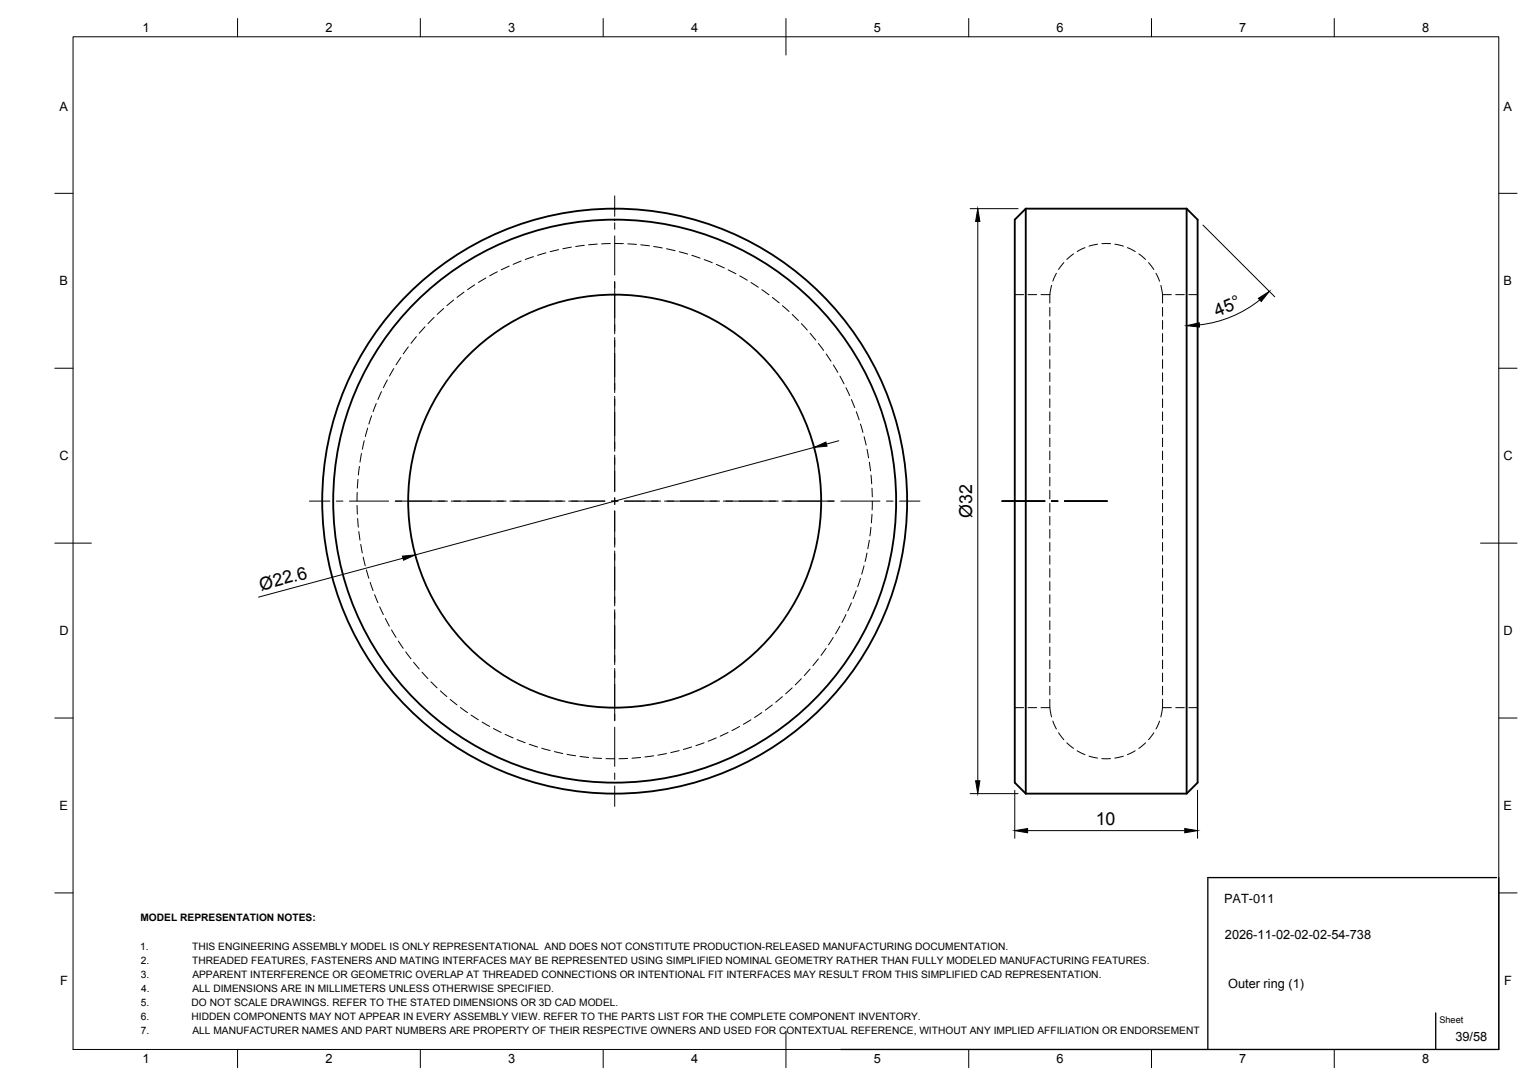
ISO-10303-21;
HEADER;
/* Generated by software containing ST-Developer
 * from STEP Tools, Inc. (www.steptools.com) 
 */

FILE_DESCRIPTION(
/* description */ ('Belt tension measurement rig'),
/* implementation_level */ '2;1');

FILE_NAME(
/* name */ 'Outer ring (1).step',
/* time_stamp */ '2026-10-28T03:24:44-07:00',
/* author */ (''),
/* organization */ (''),
/* preprocessor_version */ 'ST-DEVELOPER v20.2',
/* originating_system */ 'Autodesk Translation Framework v15.17.0.0',
/* authorisation */ '');

FILE_SCHEMA (('AUTOMOTIVE_DESIGN { 1 0 10303 214 3 1 1 }'));
ENDSEC;

DATA;
#10=MECHANICAL_DESIGN_GEOMETRIC_PRESENTATION_REPRESENTATION('',(#732),#23587);
#476=CONICAL_SURFACE('',#13686,1.57,0.785398163397449);
#477=CONICAL_SURFACE('',#13690,1.57,0.785398163397449);
#490=TOROIDAL_SURFACE('',#13675,1.1,0.309556);
#614=SHAPE_REPRESENTATION_RELATIONSHIP('SRR','None',#23863,#669);
#669=ADVANCED_BREP_SHAPE_REPRESENTATION('',(#801),#23561);
#732=STYLED_ITEM('',(#24211),#801);
#801=MANIFOLD_SOLID_BREP('Body1',#12238);
#976=FACE_BOUND('',#2597,.T.);
#977=FACE_BOUND('',#2602,.T.);
#1252=PLANE('',#13683);
#1253=PLANE('',#13692);
#1743=FACE_OUTER_BOUND('',#2594,.T.);
#1744=FACE_OUTER_BOUND('',#2595,.T.);
#1745=FACE_OUTER_BOUND('',#2596,.T.);
#1746=FACE_OUTER_BOUND('',#2598,.T.);
#1747=FACE_OUTER_BOUND('',#2599,.T.);
#1748=FACE_OUTER_BOUND('',#2600,.T.);
#1749=FACE_OUTER_BOUND('',#2601,.T.);
#1750=FACE_OUTER_BOUND('',#2603,.T.);
#2594=EDGE_LOOP('',(#9694,#9695,#9696,#9697,#9698,#9699));
#2595=EDGE_LOOP('',(#9700,#9701,#9702,#9703,#9704));
#2596=EDGE_LOOP('',(#9705));
#2597=EDGE_LOOP('',(#9706));
#2598=EDGE_LOOP('',(#9707,#9708,#9709,#9710));
#2599=EDGE_LOOP('',(#9711,#9712,#9713,#9714));
#2600=EDGE_LOOP('',(#9715,#9716,#9717,#9718));
#2601=EDGE_LOOP('',(#9719));
#2602=EDGE_LOOP('',(#9720));
#2603=EDGE_LOOP('',(#9721,#9722,#9723,#9724,#9725));
#3459=LINE('',#20899,#4210);
#3460=LINE('',#20908,#4211);
#3461=LINE('',#20912,#4212);
#3462=LINE('',#20916,#4213);
#3463=LINE('',#20919,#4214);
#4210=VECTOR('',#16622,1.129765);
#4211=VECTOR('',#16633,1.57);
#4212=VECTOR('',#16638,1.6);
#4213=VECTOR('',#16643,1.57);
#4214=VECTOR('',#16648,1.129765);
#4831=CIRCLE('',#13676,1.129765);
#4832=CIRCLE('',#13677,1.129765);
#4833=CIRCLE('',#13678,0.309556);
#4834=CIRCLE('',#13679,1.129765);
#4835=CIRCLE('',#13680,1.129765);
#4836=CIRCLE('',#13682,1.129765);
#4837=CIRCLE('',#13684,1.54);
#4838=CIRCLE('',#13685,1.129765);
#4839=CIRCLE('',#13687,1.6);
#4840=CIRCLE('',#13689,1.6);
#4841=CIRCLE('',#13691,1.54);
#5828=VERTEX_POINT('',#20887);
#5829=VERTEX_POINT('',#20888);
#5830=VERTEX_POINT('',#20891);
#5831=VERTEX_POINT('',#20893);
#5832=VERTEX_POINT('',#20897);
#5833=VERTEX_POINT('',#20901);
#5834=VERTEX_POINT('',#20903);
#5835=VERTEX_POINT('',#20906);
#5836=VERTEX_POINT('',#20910);
#5837=VERTEX_POINT('',#20914);
#7206=EDGE_CURVE('',#5828,#5829,#4831,.T.);
#7207=EDGE_CURVE('',#5829,#5828,#4832,.T.);
#7208=EDGE_CURVE('',#5829,#5830,#4833,.T.);
#7209=EDGE_CURVE('',#5831,#5830,#4834,.T.);
#7210=EDGE_CURVE('',#5830,#5831,#4835,.T.);
#7211=EDGE_CURVE('',#5832,#5832,#4836,.T.);
#7212=EDGE_CURVE('',#5832,#5831,#3459,.T.);
#7213=EDGE_CURVE('',#5833,#5833,#4837,.T.);
#7214=EDGE_CURVE('',#5834,#5834,#4838,.T.);
#7215=EDGE_CURVE('',#5835,#5835,#4839,.T.);
#7216=EDGE_CURVE('',#5835,#5833,#3460,.T.);
#7217=EDGE_CURVE('',#5836,#5836,#4840,.T.);
#7218=EDGE_CURVE('',#5836,#5835,#3461,.T.);
#7219=EDGE_CURVE('',#5837,#5837,#4841,.T.);
#7220=EDGE_CURVE('',#5837,#5836,#3462,.T.);
#7221=EDGE_CURVE('',#5828,#5834,#3463,.T.);
#9694=ORIENTED_EDGE('',*,*,#7206,.F.);
#9695=ORIENTED_EDGE('',*,*,#7207,.F.);
#9696=ORIENTED_EDGE('',*,*,#7208,.T.);
#9697=ORIENTED_EDGE('',*,*,#7209,.F.);
#9698=ORIENTED_EDGE('',*,*,#7210,.F.);
#9699=ORIENTED_EDGE('',*,*,#7208,.F.);
#9700=ORIENTED_EDGE('',*,*,#7211,.T.);
#9701=ORIENTED_EDGE('',*,*,#7212,.T.);
#9702=ORIENTED_EDGE('',*,*,#7209,.T.);
#9703=ORIENTED_EDGE('',*,*,#7210,.T.);
#9704=ORIENTED_EDGE('',*,*,#7212,.F.);
#9705=ORIENTED_EDGE('',*,*,#7213,.F.);
#9706=ORIENTED_EDGE('',*,*,#7214,.T.);
#9707=ORIENTED_EDGE('',*,*,#7215,.F.);
#9708=ORIENTED_EDGE('',*,*,#7216,.T.);
#9709=ORIENTED_EDGE('',*,*,#7213,.T.);
#9710=ORIENTED_EDGE('',*,*,#7216,.F.);
#9711=ORIENTED_EDGE('',*,*,#7217,.F.);
#9712=ORIENTED_EDGE('',*,*,#7218,.T.);
#9713=ORIENTED_EDGE('',*,*,#7215,.T.);
#9714=ORIENTED_EDGE('',*,*,#7218,.F.);
#9715=ORIENTED_EDGE('',*,*,#7219,.F.);
#9716=ORIENTED_EDGE('',*,*,#7220,.T.);
#9717=ORIENTED_EDGE('',*,*,#7217,.T.);
#9718=ORIENTED_EDGE('',*,*,#7220,.F.);
#9719=ORIENTED_EDGE('',*,*,#7219,.T.);
#9720=ORIENTED_EDGE('',*,*,#7211,.F.);
#9721=ORIENTED_EDGE('',*,*,#7206,.T.);
#9722=ORIENTED_EDGE('',*,*,#7207,.T.);
#9723=ORIENTED_EDGE('',*,*,#7221,.T.);
#9724=ORIENTED_EDGE('',*,*,#7214,.F.);
#9725=ORIENTED_EDGE('',*,*,#7221,.F.);
#11306=CYLINDRICAL_SURFACE('',#13681,1.129765);
#11307=CYLINDRICAL_SURFACE('',#13688,1.6);
#11308=CYLINDRICAL_SURFACE('',#13693,1.129765);
#11884=ADVANCED_FACE('',(#1743),#490,.F.);
#11885=ADVANCED_FACE('',(#1744),#11306,.F.);
#11886=ADVANCED_FACE('',(#1745,#976),#1252,.T.);
#11887=ADVANCED_FACE('',(#1746),#476,.T.);
#11888=ADVANCED_FACE('',(#1747),#11307,.T.);
#11889=ADVANCED_FACE('',(#1748),#477,.T.);
#11890=ADVANCED_FACE('',(#1749,#977),#1253,.T.);
#11891=ADVANCED_FACE('',(#1750),#11308,.F.);
#12238=CLOSED_SHELL('',(#11884,#11885,#11886,#11887,#11888,#11889,#11890,
#11891));
#13674=AXIS2_PLACEMENT_3D('',#20885,#16604,#16605);
#13675=AXIS2_PLACEMENT_3D('',#20886,#16606,#16607);
#13676=AXIS2_PLACEMENT_3D('',#20889,#16608,#16609);
#13677=AXIS2_PLACEMENT_3D('',#20890,#16610,#16611);
#13678=AXIS2_PLACEMENT_3D('',#20892,#16612,#16613);
#13679=AXIS2_PLACEMENT_3D('',#20894,#16614,#16615);
#13680=AXIS2_PLACEMENT_3D('',#20895,#16616,#16617);
#13681=AXIS2_PLACEMENT_3D('',#20896,#16618,#16619);
#13682=AXIS2_PLACEMENT_3D('',#20898,#16620,#16621);
#13683=AXIS2_PLACEMENT_3D('',#20900,#16623,#16624);
#13684=AXIS2_PLACEMENT_3D('',#20902,#16625,#16626);
#13685=AXIS2_PLACEMENT_3D('',#20904,#16627,#16628);
#13686=AXIS2_PLACEMENT_3D('',#20905,#16629,#16630);
#13687=AXIS2_PLACEMENT_3D('',#20907,#16631,#16632);
#13688=AXIS2_PLACEMENT_3D('',#20909,#16634,#16635);
#13689=AXIS2_PLACEMENT_3D('',#20911,#16636,#16637);
#13690=AXIS2_PLACEMENT_3D('',#20913,#16639,#16640);
#13691=AXIS2_PLACEMENT_3D('',#20915,#16641,#16642);
#13692=AXIS2_PLACEMENT_3D('',#20917,#16644,#16645);
#13693=AXIS2_PLACEMENT_3D('',#20918,#16646,#16647);
#16604=DIRECTION('axis',(0.,0.,1.));
#16605=DIRECTION('refdir',(1.,0.,0.));
#16606=DIRECTION('center_axis',(0.,-1.,0.));
#16607=DIRECTION('ref_axis',(0.,0.,-1.));
#16608=DIRECTION('center_axis',(0.,-1.,0.));
#16609=DIRECTION('ref_axis',(1.,0.,0.));
#16610=DIRECTION('center_axis',(0.,-1.,0.));
#16611=DIRECTION('ref_axis',(1.,0.,0.));
#16612=DIRECTION('center_axis',(1.,0.,1.22464679914735E-16));
#16613=DIRECTION('ref_axis',(-1.22464679914735E-16,0.,1.));
#16614=DIRECTION('center_axis',(0.,1.,0.));
#16615=DIRECTION('ref_axis',(1.,0.,0.));
#16616=DIRECTION('center_axis',(0.,1.,0.));
#16617=DIRECTION('ref_axis',(1.,0.,0.));
#16618=DIRECTION('center_axis',(0.,-1.,0.));
#16619=DIRECTION('ref_axis',(1.,0.,0.));
#16620=DIRECTION('center_axis',(0.,-1.,0.));
#16621=DIRECTION('ref_axis',(1.,0.,0.));
#16622=DIRECTION('',(0.,1.,0.));
#16623=DIRECTION('center_axis',(0.,1.,0.));
#16624=DIRECTION('ref_axis',(0.,0.,1.));
#16625=DIRECTION('center_axis',(0.,-1.,0.));
#16626=DIRECTION('ref_axis',(1.,0.,0.));
#16627=DIRECTION('center_axis',(0.,-1.,0.));
#16628=DIRECTION('ref_axis',(1.,0.,0.));
#16629=DIRECTION('center_axis',(0.,-1.,0.));
#16630=DIRECTION('ref_axis',(1.,0.,0.));
#16631=DIRECTION('center_axis',(0.,-1.,0.));
#16632=DIRECTION('ref_axis',(1.,0.,0.));
#16633=DIRECTION('',(0.707106781186548,0.707106781186547,8.65956056235494E-17));
#16634=DIRECTION('center_axis',(0.,-1.,0.));
#16635=DIRECTION('ref_axis',(1.,0.,0.));
#16636=DIRECTION('center_axis',(0.,-1.,0.));
#16637=DIRECTION('ref_axis',(1.,0.,0.));
#16638=DIRECTION('',(0.,1.,0.));
#16639=DIRECTION('center_axis',(0.,1.,0.));
#16640=DIRECTION('ref_axis',(1.,0.,0.));
#16641=DIRECTION('center_axis',(0.,-1.,0.));
#16642=DIRECTION('ref_axis',(1.,0.,0.));
#16643=DIRECTION('',(-0.707106781186548,0.707106781186547,-8.65956056235494E-17));
#16644=DIRECTION('center_axis',(0.,-1.,0.));
#16645=DIRECTION('ref_axis',(0.,0.,-1.));
#16646=DIRECTION('center_axis',(0.,-1.,0.));
#16647=DIRECTION('ref_axis',(1.,0.,0.));
#16648=DIRECTION('',(0.,1.,0.));
#20885=CARTESIAN_POINT('',(0.,0.,0.));
#20886=CARTESIAN_POINT('Origin',(0.,0.,0.));
#20887=CARTESIAN_POINT('',(-1.129765,0.308121667383195,-1.38356309103871E-16));
#20888=CARTESIAN_POINT('',(-1.38356309103871E-16,0.308121667383195,1.129765));
#20889=CARTESIAN_POINT('Origin',(0.,0.308121667383195,0.));
#20890=CARTESIAN_POINT('Origin',(0.,0.308121667383195,0.));
#20891=CARTESIAN_POINT('',(-1.38356309103871E-16,-0.308121667383195,1.129765));
#20892=CARTESIAN_POINT('Origin',(-1.34711147906209E-16,0.,1.1));
#20893=CARTESIAN_POINT('',(-1.129765,-0.308121667383195,1.38356309103871E-16));
#20894=CARTESIAN_POINT('Origin',(0.,-0.308121667383195,0.));
#20895=CARTESIAN_POINT('Origin',(0.,-0.308121667383195,0.));
#20896=CARTESIAN_POINT('Origin',(0.,0.,0.));
#20897=CARTESIAN_POINT('',(-1.129765,-0.5,-1.38356309103871E-16));
#20898=CARTESIAN_POINT('Origin',(0.,-0.5,0.));
#20899=CARTESIAN_POINT('',(-1.129765,0.,-1.38356309103871E-16));
#20900=CARTESIAN_POINT('Origin',(1.54,0.5,0.));
#20901=CARTESIAN_POINT('',(-1.54,0.5,-1.88595607068692E-16));
#20902=CARTESIAN_POINT('Origin',(0.,0.5,0.));
#20903=CARTESIAN_POINT('',(-1.129765,0.5,-1.38356309103871E-16));
#20904=CARTESIAN_POINT('Origin',(0.,0.5,0.));
#20905=CARTESIAN_POINT('Origin',(0.,0.47,0.));
#20906=CARTESIAN_POINT('',(-1.6,0.44,-1.95943487863577E-16));
#20907=CARTESIAN_POINT('Origin',(0.,0.44,0.));
#20908=CARTESIAN_POINT('',(-1.57,0.47,-1.92269547466134E-16));
#20909=CARTESIAN_POINT('Origin',(0.,0.,0.));
#20910=CARTESIAN_POINT('',(-1.6,-0.44,-1.95943487863577E-16));
#20911=CARTESIAN_POINT('Origin',(0.,-0.44,0.));
#20912=CARTESIAN_POINT('',(-1.6,0.,-1.95943487863577E-16));
#20913=CARTESIAN_POINT('Origin',(0.,-0.47,0.));
#20914=CARTESIAN_POINT('',(-1.54,-0.5,-1.88595607068692E-16));
#20915=CARTESIAN_POINT('Origin',(0.,-0.5,0.));
#20916=CARTESIAN_POINT('',(-1.57,-0.47,-1.92269547466134E-16));
#20917=CARTESIAN_POINT('Origin',(1.129765,-0.5,0.));
#20918=CARTESIAN_POINT('Origin',(0.,0.,0.));
#20919=CARTESIAN_POINT('',(-1.129765,0.,-1.38356309103871E-16));
#23496=UNCERTAINTY_MEASURE_WITH_UNIT(LENGTH_MEASURE(0.001),#23588,
'DISTANCE_ACCURACY_VALUE',
'Maximum model space distance between geometric entities at asserted c
onnectivities');
#23522=UNCERTAINTY_MEASURE_WITH_UNIT(LENGTH_MEASURE(0.001),#23588,
'DISTANCE_ACCURACY_VALUE',
'Maximum model space distance between geometric entities at asserted c
onnectivities');
#23561=(
GEOMETRIC_REPRESENTATION_CONTEXT(3)
GLOBAL_UNCERTAINTY_ASSIGNED_CONTEXT((#23496))
GLOBAL_UNIT_ASSIGNED_CONTEXT((#23588,#23590,#23591))
REPRESENTATION_CONTEXT('','3D')
);
#23587=(
GEOMETRIC_REPRESENTATION_CONTEXT(3)
GLOBAL_UNCERTAINTY_ASSIGNED_CONTEXT((#23522))
GLOBAL_UNIT_ASSIGNED_CONTEXT((#23588,#23590,#23591))
REPRESENTATION_CONTEXT('','3D')
);
#23588=(
LENGTH_UNIT()
NAMED_UNIT(*)
SI_UNIT(.CENTI.,.METRE.)
);
#23590=(
NAMED_UNIT(*)
PLANE_ANGLE_UNIT()
SI_UNIT($,.RADIAN.)
);
#23591=(
NAMED_UNIT(*)
SI_UNIT($,.STERADIAN.)
SOLID_ANGLE_UNIT()
);
#23630=SHAPE_DEFINITION_REPRESENTATION(#23702,#23863);
#23702=PRODUCT_DEFINITION_SHAPE('',$,#23928);
#23863=SHAPE_REPRESENTATION('',(#13674),#23561);
#23889=PRODUCT_DEFINITION_CONTEXT('part definition',#24083,'design');
#23928=PRODUCT_DEFINITION('Outer ring (1)','Outer ring (1)',#23992,#23889);
#23992=PRODUCT_DEFINITION_FORMATION('',$,#24123);
#24083=APPLICATION_CONTEXT(
'Core Data for Automotive Mechanical Design Process');
#24084=PRODUCT_CONTEXT('part definition',#24083,'mechanical');
#24123=PRODUCT('Outer ring (1)','Outer ring (1)','Outer ring (1)',(#24084));
#24205=COLOUR_RGB('Grey',0.48,0.52,0.57);
#24206=FILL_AREA_STYLE_COLOUR('',#24205);
#24207=FILL_AREA_STYLE('',(#24206));
#24208=SURFACE_STYLE_FILL_AREA(#24207);
#24209=SURFACE_SIDE_STYLE('',(#24208));
#24210=SURFACE_STYLE_USAGE(.BOTH.,#24209);
#24211=PRESENTATION_STYLE_ASSIGNMENT((#24210));
ENDSEC;
END-ISO-10303-21;
